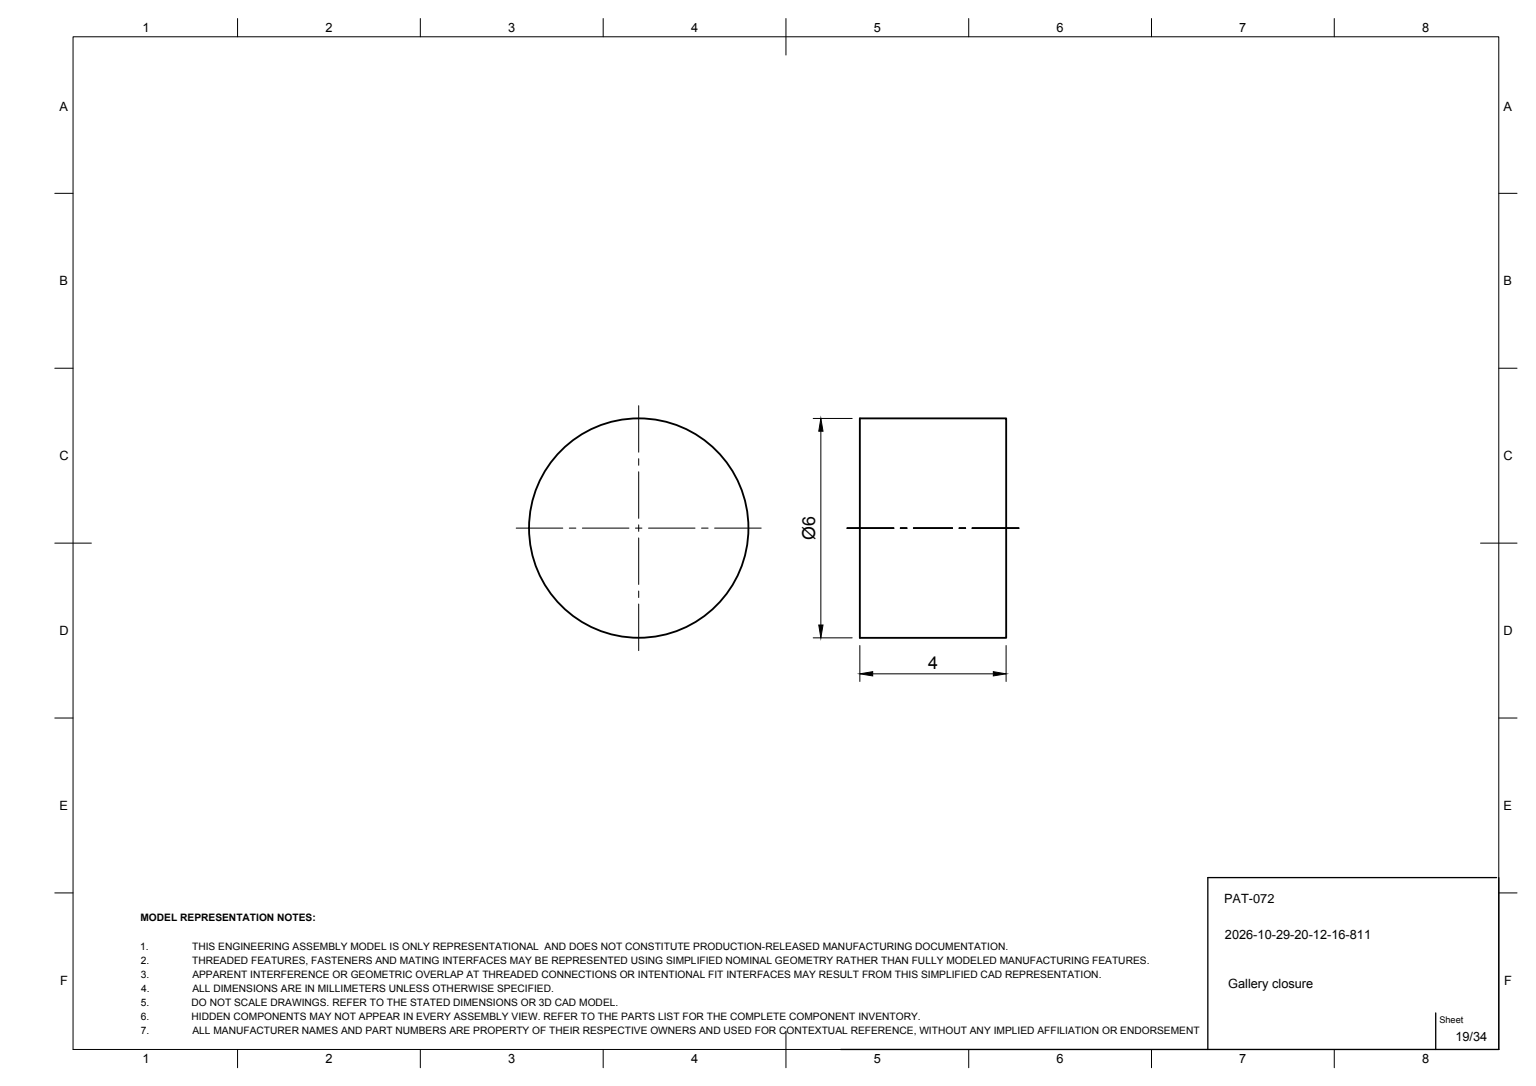
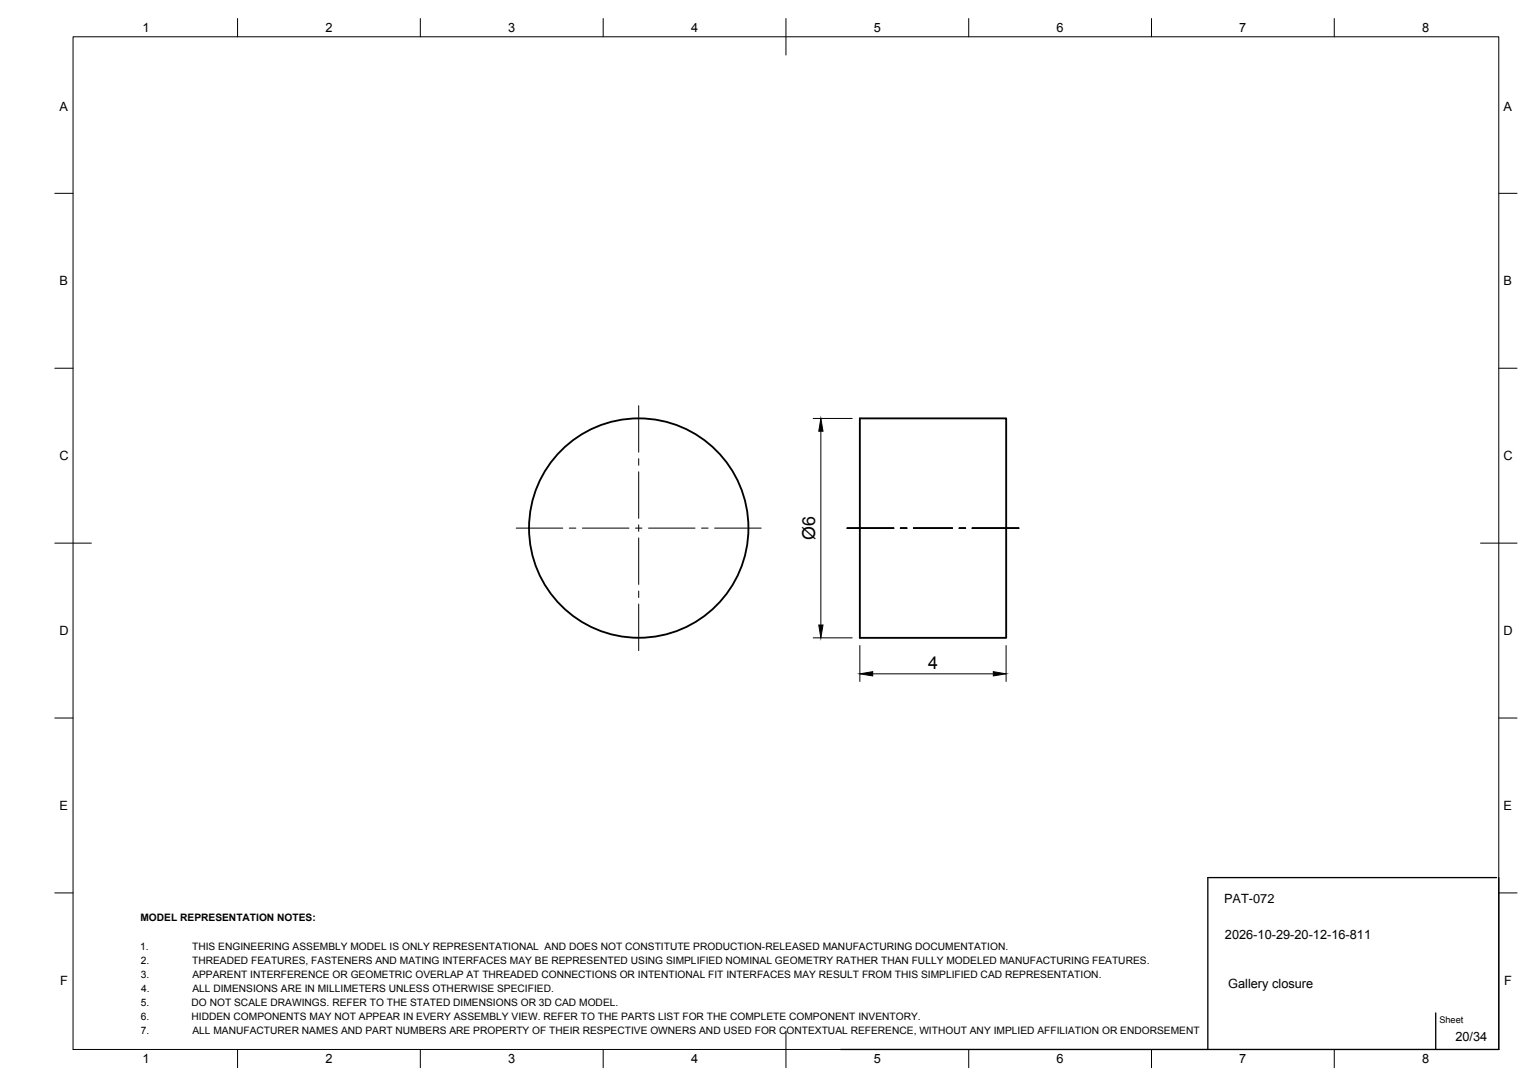
ISO-10303-21;
HEADER;
/* Generated by software containing ST-Developer
 * from STEP Tools, Inc. (www.steptools.com) 
 */

FILE_DESCRIPTION(
/* description */ ('PAT-072'),
/* implementation_level */ '2;1');

FILE_NAME(
/* name */ 'Gallery closure.step',
/* time_stamp */ '2026-10-29T20:11:56-07:00',
/* author */ (''),
/* organization */ (''),
/* preprocessor_version */ 'ST-DEVELOPER v20.2',
/* originating_system */ 'Autodesk Translation Framework v15.17.0.0',
/* authorisation */ '');

FILE_SCHEMA (('AUTOMOTIVE_DESIGN { 1 0 10303 214 3 1 1 }'));
ENDSEC;

DATA;
#10=MECHANICAL_DESIGN_GEOMETRIC_PRESENTATION_REPRESENTATION('',(#348),#11432);
#276=SHAPE_REPRESENTATION_RELATIONSHIP('SRR','None',#11580,#312);
#312=ADVANCED_BREP_SHAPE_REPRESENTATION('',(#384),#11411);
#348=STYLED_ITEM('',(#11812),#384);
#384=MANIFOLD_SOLID_BREP('Body1',#6083);
#653=PLANE('',#6824);
#654=PLANE('',#6825);
#953=FACE_OUTER_BOUND('',#1407,.T.);
#954=FACE_OUTER_BOUND('',#1408,.T.);
#955=FACE_OUTER_BOUND('',#1409,.T.);
#1407=EDGE_LOOP('',(#4666,#4667,#4668,#4669));
#1408=EDGE_LOOP('',(#4670));
#1409=EDGE_LOOP('',(#4671));
#1838=LINE('',#10205,#2257);
#2257=VECTOR('',#8031,0.3);
#2683=CIRCLE('',#6822,0.3);
#2684=CIRCLE('',#6823,0.3);
#3032=VERTEX_POINT('',#10202);
#3033=VERTEX_POINT('',#10204);
#3622=EDGE_CURVE('',#3032,#3032,#2683,.T.);
#3623=EDGE_CURVE('',#3032,#3033,#1838,.T.);
#3624=EDGE_CURVE('',#3033,#3033,#2684,.T.);
#4666=ORIENTED_EDGE('',*,*,#3622,.F.);
#4667=ORIENTED_EDGE('',*,*,#3623,.T.);
#4668=ORIENTED_EDGE('',*,*,#3624,.T.);
#4669=ORIENTED_EDGE('',*,*,#3623,.F.);
#4670=ORIENTED_EDGE('',*,*,#3622,.T.);
#4671=ORIENTED_EDGE('',*,*,#3624,.F.);
#5632=CYLINDRICAL_SURFACE('',#6821,0.3);
#5852=ADVANCED_FACE('',(#953),#5632,.T.);
#5853=ADVANCED_FACE('',(#954),#653,.T.);
#5854=ADVANCED_FACE('',(#955),#654,.F.);
#6083=CLOSED_SHELL('',(#5852,#5853,#5854));
#6820=AXIS2_PLACEMENT_3D('',#10200,#8025,#8026);
#6821=AXIS2_PLACEMENT_3D('',#10201,#8027,#8028);
#6822=AXIS2_PLACEMENT_3D('',#10203,#8029,#8030);
#6823=AXIS2_PLACEMENT_3D('',#10206,#8032,#8033);
#6824=AXIS2_PLACEMENT_3D('',#10207,#8034,#8035);
#6825=AXIS2_PLACEMENT_3D('',#10208,#8036,#8037);
#8025=DIRECTION('axis',(0.,0.,1.));
#8026=DIRECTION('refdir',(1.,0.,0.));
#8027=DIRECTION('center_axis',(1.,0.,0.));
#8028=DIRECTION('ref_axis',(0.,0.,-1.));
#8029=DIRECTION('center_axis',(1.,0.,0.));
#8030=DIRECTION('ref_axis',(0.,0.,-1.));
#8031=DIRECTION('',(-1.,0.,0.));
#8032=DIRECTION('center_axis',(1.,0.,0.));
#8033=DIRECTION('ref_axis',(0.,0.,-1.));
#8034=DIRECTION('center_axis',(1.,0.,0.));
#8035=DIRECTION('ref_axis',(0.,0.,-1.));
#8036=DIRECTION('center_axis',(1.,0.,0.));
#8037=DIRECTION('ref_axis',(0.,0.,-1.));
#10200=CARTESIAN_POINT('',(0.,0.,0.));
#10201=CARTESIAN_POINT('Origin',(-5.5,1.5,4.));
#10202=CARTESIAN_POINT('',(-5.1,1.5,4.3));
#10203=CARTESIAN_POINT('Origin',(-5.1,1.5,4.));
#10204=CARTESIAN_POINT('',(-5.5,1.5,4.3));
#10205=CARTESIAN_POINT('',(-5.5,1.5,4.3));
#10206=CARTESIAN_POINT('Origin',(-5.5,1.5,4.));
#10207=CARTESIAN_POINT('Origin',(-5.1,1.5,4.));
#10208=CARTESIAN_POINT('Origin',(-5.5,1.5,4.));
#11372=UNCERTAINTY_MEASURE_WITH_UNIT(LENGTH_MEASURE(0.001),#11433,
'DISTANCE_ACCURACY_VALUE',
'Maximum model space distance between geometric entities at asserted c
onnectivities');
#11393=UNCERTAINTY_MEASURE_WITH_UNIT(LENGTH_MEASURE(0.001),#11433,
'DISTANCE_ACCURACY_VALUE',
'Maximum model space distance between geometric entities at asserted c
onnectivities');
#11411=(
GEOMETRIC_REPRESENTATION_CONTEXT(3)
GLOBAL_UNCERTAINTY_ASSIGNED_CONTEXT((#11372))
GLOBAL_UNIT_ASSIGNED_CONTEXT((#11433,#11435,#11436))
REPRESENTATION_CONTEXT('','3D')
);
#11432=(
GEOMETRIC_REPRESENTATION_CONTEXT(3)
GLOBAL_UNCERTAINTY_ASSIGNED_CONTEXT((#11393))
GLOBAL_UNIT_ASSIGNED_CONTEXT((#11433,#11435,#11436))
REPRESENTATION_CONTEXT('','3D')
);
#11433=(
LENGTH_UNIT()
NAMED_UNIT(*)
SI_UNIT(.CENTI.,.METRE.)
);
#11435=(
NAMED_UNIT(*)
PLANE_ANGLE_UNIT()
SI_UNIT($,.RADIAN.)
);
#11436=(
NAMED_UNIT(*)
SI_UNIT($,.STERADIAN.)
SOLID_ANGLE_UNIT()
);
#11454=SHAPE_DEFINITION_REPRESENTATION(#11492,#11580);
#11492=PRODUCT_DEFINITION_SHAPE('',$,#11619);
#11580=SHAPE_REPRESENTATION('',(#6820),#11411);
#11601=PRODUCT_DEFINITION_CONTEXT('part definition',#11717,'design');
#11619=PRODUCT_DEFINITION('Gallery closure','Gallery closure',
#11657,#11601);
#11657=PRODUCT_DEFINITION_FORMATION('',$,#11736);
#11717=APPLICATION_CONTEXT(
'Core Data for Automotive Mechanical Design Process');
#11718=PRODUCT_CONTEXT('part definition',#11717,'mechanical');
#11736=PRODUCT('Gallery closure','Gallery closure',
'Gallery closure',(#11718));
#11806=COLOUR_RGB('Sky Blue',0.24,0.69,0.87);
#11807=FILL_AREA_STYLE_COLOUR('',#11806);
#11808=FILL_AREA_STYLE('',(#11807));
#11809=SURFACE_STYLE_FILL_AREA(#11808);
#11810=SURFACE_SIDE_STYLE('',(#11809));
#11811=SURFACE_STYLE_USAGE(.BOTH.,#11810);
#11812=PRESENTATION_STYLE_ASSIGNMENT((#11811));
ENDSEC;
END-ISO-10303-21;
